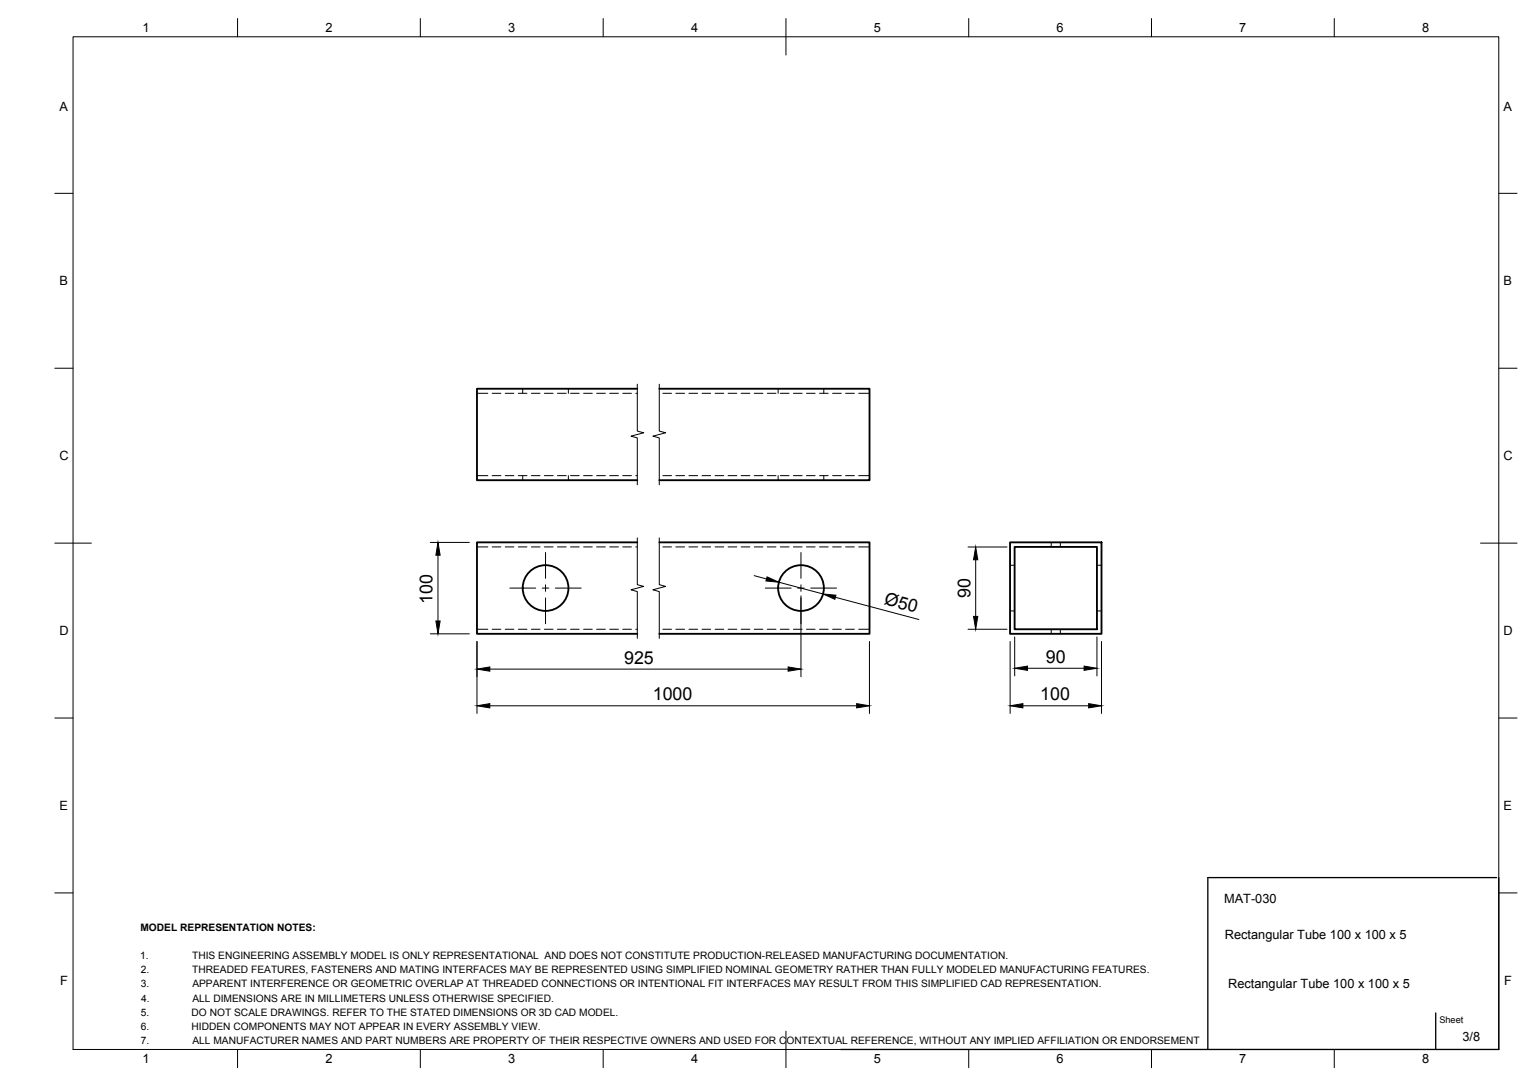
ISO-10303-21;
HEADER;
/* Generated by software containing ST-Developer
 * from STEP Tools, Inc. (www.steptools.com) 
 */

FILE_DESCRIPTION(
/* description */ ('STEP AP214'),
/* implementation_level */ '2;1');

FILE_NAME(
/* name */ 'Rectangular Tube 100 x 100 x 5.step',
/* time_stamp */ '2026-11-14T06:43:04-08:00',
/* author */ (''),
/* organization */ (''),
/* preprocessor_version */ 'ST-DEVELOPER v20.2',
/* originating_system */ 'Autodesk Translation Framework v15.17.0.0',
/* authorisation */ '');

FILE_SCHEMA (('AUTOMOTIVE_DESIGN { 1 0 10303 214 3 1 1 }'));
ENDSEC;

DATA;
#10=MECHANICAL_DESIGN_GEOMETRIC_PRESENTATION_REPRESENTATION('',(#204),#5658);
#182=SHAPE_REPRESENTATION_RELATIONSHIP('SRR','None',#5712,#193);
#193=ADVANCED_BREP_SHAPE_REPRESENTATION('',(#215),#5653);
#204=STYLED_ITEM('',(#5772),#215);
#215=MANIFOLD_SOLID_BREP('Body1',#3066);
#254=CYLINDRICAL_SURFACE('',#3398,5.);
#255=CYLINDRICAL_SURFACE('',#3401,5.);
#256=CYLINDRICAL_SURFACE('',#3404,5.);
#257=CYLINDRICAL_SURFACE('',#3407,5.);
#258=CYLINDRICAL_SURFACE('',#3410,25.);
#259=CYLINDRICAL_SURFACE('',#3413,25.);
#260=CYLINDRICAL_SURFACE('',#3416,25.);
#261=CYLINDRICAL_SURFACE('',#3419,25.);
#311=FACE_BOUND('',#675,.T.);
#312=FACE_BOUND('',#677,.T.);
#313=FACE_BOUND('',#679,.T.);
#314=FACE_BOUND('',#680,.T.);
#315=FACE_BOUND('',#682,.T.);
#316=FACE_BOUND('',#683,.T.);
#317=FACE_BOUND('',#685,.T.);
#318=FACE_BOUND('',#686,.T.);
#319=FACE_BOUND('',#688,.T.);
#320=FACE_BOUND('',#689,.T.);
#321=FACE_BOUND('',#691,.T.);
#322=FACE_BOUND('',#692,.T.);
#323=FACE_BOUND('',#694,.T.);
#324=FACE_BOUND('',#695,.T.);
#325=FACE_BOUND('',#697,.T.);
#326=FACE_BOUND('',#698,.T.);
#327=FACE_BOUND('',#700,.T.);
#328=FACE_BOUND('',#701,.T.);
#444=FACE_OUTER_BOUND('',#666,.T.);
#445=FACE_OUTER_BOUND('',#667,.T.);
#446=FACE_OUTER_BOUND('',#668,.T.);
#447=FACE_OUTER_BOUND('',#669,.T.);
#448=FACE_OUTER_BOUND('',#670,.T.);
#449=FACE_OUTER_BOUND('',#671,.T.);
#450=FACE_OUTER_BOUND('',#672,.T.);
#451=FACE_OUTER_BOUND('',#673,.T.);
#452=FACE_OUTER_BOUND('',#674,.T.);
#453=FACE_OUTER_BOUND('',#676,.T.);
#454=FACE_OUTER_BOUND('',#678,.T.);
#455=FACE_OUTER_BOUND('',#681,.T.);
#456=FACE_OUTER_BOUND('',#684,.T.);
#457=FACE_OUTER_BOUND('',#687,.T.);
#458=FACE_OUTER_BOUND('',#690,.T.);
#459=FACE_OUTER_BOUND('',#693,.T.);
#460=FACE_OUTER_BOUND('',#696,.T.);
#461=FACE_OUTER_BOUND('',#699,.T.);
#666=EDGE_LOOP('',(#2460,#2461,#2462,#2463));
#667=EDGE_LOOP('',(#2464,#2465,#2466,#2467));
#668=EDGE_LOOP('',(#2468,#2469,#2470,#2471));
#669=EDGE_LOOP('',(#2472,#2473,#2474,#2475));
#670=EDGE_LOOP('',(#2476,#2477,#2478,#2479));
#671=EDGE_LOOP('',(#2480,#2481,#2482,#2483));
#672=EDGE_LOOP('',(#2484,#2485,#2486,#2487));
#673=EDGE_LOOP('',(#2488,#2489,#2490,#2491));
#674=EDGE_LOOP('',(#2492,#2493,#2494,#2495));
#675=EDGE_LOOP('',(#2496,#2497,#2498,#2499));
#676=EDGE_LOOP('',(#2500,#2501,#2502,#2503));
#677=EDGE_LOOP('',(#2504,#2505,#2506,#2507));
#678=EDGE_LOOP('',(#2508,#2509,#2510,#2511));
#679=EDGE_LOOP('',(#2512));
#680=EDGE_LOOP('',(#2513));
#681=EDGE_LOOP('',(#2514,#2515,#2516,#2517));
#682=EDGE_LOOP('',(#2518));
#683=EDGE_LOOP('',(#2519));
#684=EDGE_LOOP('',(#2520,#2521,#2522,#2523));
#685=EDGE_LOOP('',(#2524));
#686=EDGE_LOOP('',(#2525));
#687=EDGE_LOOP('',(#2526,#2527,#2528,#2529));
#688=EDGE_LOOP('',(#2530));
#689=EDGE_LOOP('',(#2531));
#690=EDGE_LOOP('',(#2532,#2533,#2534,#2535));
#691=EDGE_LOOP('',(#2536));
#692=EDGE_LOOP('',(#2537));
#693=EDGE_LOOP('',(#2538,#2539,#2540,#2541));
#694=EDGE_LOOP('',(#2542));
#695=EDGE_LOOP('',(#2543));
#696=EDGE_LOOP('',(#2544,#2545,#2546,#2547));
#697=EDGE_LOOP('',(#2548));
#698=EDGE_LOOP('',(#2549));
#699=EDGE_LOOP('',(#2550,#2551,#2552,#2553));
#700=EDGE_LOOP('',(#2554));
#701=EDGE_LOOP('',(#2555));
#864=LINE('',#5273,#1060);
#865=LINE('',#5279,#1061);
#866=LINE('',#5285,#1062);
#867=LINE('',#5291,#1063);
#868=LINE('',#5297,#1064);
#869=LINE('',#5303,#1065);
#870=LINE('',#5309,#1066);
#871=LINE('',#5315,#1067);
#872=LINE('',#5320,#1068);
#873=LINE('',#5322,#1069);
#874=LINE('',#5324,#1070);
#875=LINE('',#5325,#1071);
#876=LINE('',#5328,#1072);
#877=LINE('',#5330,#1073);
#878=LINE('',#5332,#1074);
#879=LINE('',#5333,#1075);
#880=LINE('',#5337,#1076);
#881=LINE('',#5339,#1077);
#882=LINE('',#5341,#1078);
#883=LINE('',#5342,#1079);
#884=LINE('',#5345,#1080);
#885=LINE('',#5347,#1081);
#886=LINE('',#5349,#1082);
#887=LINE('',#5350,#1083);
#888=LINE('',#5352,#1084);
#889=LINE('',#5353,#1085);
#890=LINE('',#5355,#1086);
#891=LINE('',#5357,#1087);
#892=LINE('',#5360,#1088);
#893=LINE('',#5361,#1089);
#894=LINE('',#5363,#1090);
#895=LINE('',#5365,#1091);
#1060=VECTOR('',#4070,5.);
#1061=VECTOR('',#4077,5.);
#1062=VECTOR('',#4084,5.);
#1063=VECTOR('',#4091,5.);
#1064=VECTOR('',#4098,25.);
#1065=VECTOR('',#4105,25.);
#1066=VECTOR('',#4112,25.);
#1067=VECTOR('',#4119,25.);
#1068=VECTOR('',#4124,1000.);
#1069=VECTOR('',#4125,1000.);
#1070=VECTOR('',#4126,1000.);
#1071=VECTOR('',#4127,1000.);
#1072=VECTOR('',#4128,1000.);
#1073=VECTOR('',#4129,1000.);
#1074=VECTOR('',#4130,1000.);
#1075=VECTOR('',#4131,1000.);
#1076=VECTOR('',#4134,1000.);
#1077=VECTOR('',#4135,1000.);
#1078=VECTOR('',#4136,1000.);
#1079=VECTOR('',#4137,1000.);
#1080=VECTOR('',#4138,1000.);
#1081=VECTOR('',#4139,1000.);
#1082=VECTOR('',#4140,1000.);
#1083=VECTOR('',#4141,1000.);
#1084=VECTOR('',#4144,1000.);
#1085=VECTOR('',#4145,1000.);
#1086=VECTOR('',#4148,1000.);
#1087=VECTOR('',#4151,1000.);
#1088=VECTOR('',#4156,1000.);
#1089=VECTOR('',#4157,1000.);
#1090=VECTOR('',#4160,1000.);
#1091=VECTOR('',#4163,1000.);
#1250=CIRCLE('',#3399,5.);
#1251=CIRCLE('',#3400,5.);
#1252=CIRCLE('',#3402,5.);
#1253=CIRCLE('',#3403,5.);
#1254=CIRCLE('',#3405,5.);
#1255=CIRCLE('',#3406,5.);
#1256=CIRCLE('',#3408,5.);
#1257=CIRCLE('',#3409,5.);
#1258=CIRCLE('',#3411,25.);
#1259=CIRCLE('',#3412,25.);
#1260=CIRCLE('',#3414,25.);
#1261=CIRCLE('',#3415,25.);
#1262=CIRCLE('',#3417,25.);
#1263=CIRCLE('',#3418,25.);
#1264=CIRCLE('',#3420,25.);
#1265=CIRCLE('',#3421,25.);
#1467=VERTEX_POINT('',#5270);
#1468=VERTEX_POINT('',#5272);
#1469=VERTEX_POINT('',#5276);
#1470=VERTEX_POINT('',#5278);
#1471=VERTEX_POINT('',#5282);
#1472=VERTEX_POINT('',#5284);
#1473=VERTEX_POINT('',#5288);
#1474=VERTEX_POINT('',#5290);
#1475=VERTEX_POINT('',#5294);
#1476=VERTEX_POINT('',#5296);
#1477=VERTEX_POINT('',#5300);
#1478=VERTEX_POINT('',#5302);
#1479=VERTEX_POINT('',#5306);
#1480=VERTEX_POINT('',#5308);
#1481=VERTEX_POINT('',#5312);
#1482=VERTEX_POINT('',#5314);
#1483=VERTEX_POINT('',#5318);
#1484=VERTEX_POINT('',#5319);
#1485=VERTEX_POINT('',#5321);
#1486=VERTEX_POINT('',#5323);
#1487=VERTEX_POINT('',#5326);
#1488=VERTEX_POINT('',#5327);
#1489=VERTEX_POINT('',#5329);
#1490=VERTEX_POINT('',#5331);
#1491=VERTEX_POINT('',#5335);
#1492=VERTEX_POINT('',#5336);
#1493=VERTEX_POINT('',#5338);
#1494=VERTEX_POINT('',#5340);
#1495=VERTEX_POINT('',#5343);
#1496=VERTEX_POINT('',#5344);
#1497=VERTEX_POINT('',#5346);
#1498=VERTEX_POINT('',#5348);
#1813=EDGE_CURVE('',#1467,#1467,#1250,.T.);
#1814=EDGE_CURVE('',#1467,#1468,#864,.T.);
#1815=EDGE_CURVE('',#1468,#1468,#1251,.T.);
#1816=EDGE_CURVE('',#1469,#1469,#1252,.T.);
#1817=EDGE_CURVE('',#1469,#1470,#865,.T.);
#1818=EDGE_CURVE('',#1470,#1470,#1253,.T.);
#1819=EDGE_CURVE('',#1471,#1471,#1254,.T.);
#1820=EDGE_CURVE('',#1471,#1472,#866,.T.);
#1821=EDGE_CURVE('',#1472,#1472,#1255,.T.);
#1822=EDGE_CURVE('',#1473,#1473,#1256,.T.);
#1823=EDGE_CURVE('',#1473,#1474,#867,.T.);
#1824=EDGE_CURVE('',#1474,#1474,#1257,.T.);
#1825=EDGE_CURVE('',#1475,#1475,#1258,.T.);
#1826=EDGE_CURVE('',#1475,#1476,#868,.T.);
#1827=EDGE_CURVE('',#1476,#1476,#1259,.T.);
#1828=EDGE_CURVE('',#1477,#1477,#1260,.T.);
#1829=EDGE_CURVE('',#1477,#1478,#869,.T.);
#1830=EDGE_CURVE('',#1478,#1478,#1261,.T.);
#1831=EDGE_CURVE('',#1479,#1479,#1262,.T.);
#1832=EDGE_CURVE('',#1479,#1480,#870,.T.);
#1833=EDGE_CURVE('',#1480,#1480,#1263,.T.);
#1834=EDGE_CURVE('',#1481,#1481,#1264,.T.);
#1835=EDGE_CURVE('',#1481,#1482,#871,.T.);
#1836=EDGE_CURVE('',#1482,#1482,#1265,.T.);
#1837=EDGE_CURVE('',#1483,#1484,#872,.T.);
#1838=EDGE_CURVE('',#1484,#1485,#873,.T.);
#1839=EDGE_CURVE('',#1486,#1485,#874,.T.);
#1840=EDGE_CURVE('',#1483,#1486,#875,.T.);
#1841=EDGE_CURVE('',#1487,#1488,#876,.T.);
#1842=EDGE_CURVE('',#1489,#1487,#877,.T.);
#1843=EDGE_CURVE('',#1489,#1490,#878,.T.);
#1844=EDGE_CURVE('',#1490,#1488,#879,.T.);
#1845=EDGE_CURVE('',#1491,#1492,#880,.T.);
#1846=EDGE_CURVE('',#1491,#1493,#881,.T.);
#1847=EDGE_CURVE('',#1493,#1494,#882,.T.);
#1848=EDGE_CURVE('',#1492,#1494,#883,.T.);
#1849=EDGE_CURVE('',#1495,#1496,#884,.T.);
#1850=EDGE_CURVE('',#1496,#1497,#885,.T.);
#1851=EDGE_CURVE('',#1498,#1497,#886,.T.);
#1852=EDGE_CURVE('',#1495,#1498,#887,.T.);
#1853=EDGE_CURVE('',#1484,#1492,#888,.T.);
#1854=EDGE_CURVE('',#1483,#1491,#889,.T.);
#1855=EDGE_CURVE('',#1485,#1494,#890,.T.);
#1856=EDGE_CURVE('',#1486,#1493,#891,.T.);
#1857=EDGE_CURVE('',#1489,#1495,#892,.T.);
#1858=EDGE_CURVE('',#1487,#1496,#893,.T.);
#1859=EDGE_CURVE('',#1488,#1497,#894,.T.);
#1860=EDGE_CURVE('',#1490,#1498,#895,.T.);
#2460=ORIENTED_EDGE('',*,*,#1813,.F.);
#2461=ORIENTED_EDGE('',*,*,#1814,.T.);
#2462=ORIENTED_EDGE('',*,*,#1815,.T.);
#2463=ORIENTED_EDGE('',*,*,#1814,.F.);
#2464=ORIENTED_EDGE('',*,*,#1816,.F.);
#2465=ORIENTED_EDGE('',*,*,#1817,.T.);
#2466=ORIENTED_EDGE('',*,*,#1818,.T.);
#2467=ORIENTED_EDGE('',*,*,#1817,.F.);
#2468=ORIENTED_EDGE('',*,*,#1819,.F.);
#2469=ORIENTED_EDGE('',*,*,#1820,.T.);
#2470=ORIENTED_EDGE('',*,*,#1821,.T.);
#2471=ORIENTED_EDGE('',*,*,#1820,.F.);
#2472=ORIENTED_EDGE('',*,*,#1822,.F.);
#2473=ORIENTED_EDGE('',*,*,#1823,.T.);
#2474=ORIENTED_EDGE('',*,*,#1824,.T.);
#2475=ORIENTED_EDGE('',*,*,#1823,.F.);
#2476=ORIENTED_EDGE('',*,*,#1825,.T.);
#2477=ORIENTED_EDGE('',*,*,#1826,.T.);
#2478=ORIENTED_EDGE('',*,*,#1827,.T.);
#2479=ORIENTED_EDGE('',*,*,#1826,.F.);
#2480=ORIENTED_EDGE('',*,*,#1828,.T.);
#2481=ORIENTED_EDGE('',*,*,#1829,.T.);
#2482=ORIENTED_EDGE('',*,*,#1830,.T.);
#2483=ORIENTED_EDGE('',*,*,#1829,.F.);
#2484=ORIENTED_EDGE('',*,*,#1831,.F.);
#2485=ORIENTED_EDGE('',*,*,#1832,.T.);
#2486=ORIENTED_EDGE('',*,*,#1833,.F.);
#2487=ORIENTED_EDGE('',*,*,#1832,.F.);
#2488=ORIENTED_EDGE('',*,*,#1834,.F.);
#2489=ORIENTED_EDGE('',*,*,#1835,.T.);
#2490=ORIENTED_EDGE('',*,*,#1836,.F.);
#2491=ORIENTED_EDGE('',*,*,#1835,.F.);
#2492=ORIENTED_EDGE('',*,*,#1837,.T.);
#2493=ORIENTED_EDGE('',*,*,#1838,.T.);
#2494=ORIENTED_EDGE('',*,*,#1839,.F.);
#2495=ORIENTED_EDGE('',*,*,#1840,.F.);
#2496=ORIENTED_EDGE('',*,*,#1841,.F.);
#2497=ORIENTED_EDGE('',*,*,#1842,.F.);
#2498=ORIENTED_EDGE('',*,*,#1843,.T.);
#2499=ORIENTED_EDGE('',*,*,#1844,.T.);
#2500=ORIENTED_EDGE('',*,*,#1845,.F.);
#2501=ORIENTED_EDGE('',*,*,#1846,.T.);
#2502=ORIENTED_EDGE('',*,*,#1847,.T.);
#2503=ORIENTED_EDGE('',*,*,#1848,.F.);
#2504=ORIENTED_EDGE('',*,*,#1849,.T.);
#2505=ORIENTED_EDGE('',*,*,#1850,.T.);
#2506=ORIENTED_EDGE('',*,*,#1851,.F.);
#2507=ORIENTED_EDGE('',*,*,#1852,.F.);
#2508=ORIENTED_EDGE('',*,*,#1845,.T.);
#2509=ORIENTED_EDGE('',*,*,#1853,.F.);
#2510=ORIENTED_EDGE('',*,*,#1837,.F.);
#2511=ORIENTED_EDGE('',*,*,#1854,.T.);
#2512=ORIENTED_EDGE('',*,*,#1827,.F.);
#2513=ORIENTED_EDGE('',*,*,#1830,.F.);
#2514=ORIENTED_EDGE('',*,*,#1848,.T.);
#2515=ORIENTED_EDGE('',*,*,#1855,.F.);
#2516=ORIENTED_EDGE('',*,*,#1838,.F.);
#2517=ORIENTED_EDGE('',*,*,#1853,.T.);
#2518=ORIENTED_EDGE('',*,*,#1813,.T.);
#2519=ORIENTED_EDGE('',*,*,#1816,.T.);
#2520=ORIENTED_EDGE('',*,*,#1847,.F.);
#2521=ORIENTED_EDGE('',*,*,#1856,.F.);
#2522=ORIENTED_EDGE('',*,*,#1839,.T.);
#2523=ORIENTED_EDGE('',*,*,#1855,.T.);
#2524=ORIENTED_EDGE('',*,*,#1831,.T.);
#2525=ORIENTED_EDGE('',*,*,#1834,.T.);
#2526=ORIENTED_EDGE('',*,*,#1846,.F.);
#2527=ORIENTED_EDGE('',*,*,#1854,.F.);
#2528=ORIENTED_EDGE('',*,*,#1840,.T.);
#2529=ORIENTED_EDGE('',*,*,#1856,.T.);
#2530=ORIENTED_EDGE('',*,*,#1821,.F.);
#2531=ORIENTED_EDGE('',*,*,#1824,.F.);
#2532=ORIENTED_EDGE('',*,*,#1849,.F.);
#2533=ORIENTED_EDGE('',*,*,#1857,.F.);
#2534=ORIENTED_EDGE('',*,*,#1842,.T.);
#2535=ORIENTED_EDGE('',*,*,#1858,.T.);
#2536=ORIENTED_EDGE('',*,*,#1825,.F.);
#2537=ORIENTED_EDGE('',*,*,#1828,.F.);
#2538=ORIENTED_EDGE('',*,*,#1850,.F.);
#2539=ORIENTED_EDGE('',*,*,#1858,.F.);
#2540=ORIENTED_EDGE('',*,*,#1841,.T.);
#2541=ORIENTED_EDGE('',*,*,#1859,.T.);
#2542=ORIENTED_EDGE('',*,*,#1815,.F.);
#2543=ORIENTED_EDGE('',*,*,#1818,.F.);
#2544=ORIENTED_EDGE('',*,*,#1851,.T.);
#2545=ORIENTED_EDGE('',*,*,#1859,.F.);
#2546=ORIENTED_EDGE('',*,*,#1844,.F.);
#2547=ORIENTED_EDGE('',*,*,#1860,.T.);
#2548=ORIENTED_EDGE('',*,*,#1833,.T.);
#2549=ORIENTED_EDGE('',*,*,#1836,.T.);
#2550=ORIENTED_EDGE('',*,*,#1852,.T.);
#2551=ORIENTED_EDGE('',*,*,#1860,.F.);
#2552=ORIENTED_EDGE('',*,*,#1843,.F.);
#2553=ORIENTED_EDGE('',*,*,#1857,.T.);
#2554=ORIENTED_EDGE('',*,*,#1819,.T.);
#2555=ORIENTED_EDGE('',*,*,#1822,.T.);
#2832=PLANE('',#3422);
#2833=PLANE('',#3423);
#2834=PLANE('',#3424);
#2835=PLANE('',#3425);
#2836=PLANE('',#3426);
#2837=PLANE('',#3427);
#2838=PLANE('',#3428);
#2839=PLANE('',#3429);
#2840=PLANE('',#3430);
#2841=PLANE('',#3431);
#2985=ADVANCED_FACE('',(#444),#254,.F.);
#2986=ADVANCED_FACE('',(#445),#255,.F.);
#2987=ADVANCED_FACE('',(#446),#256,.F.);
#2988=ADVANCED_FACE('',(#447),#257,.F.);
#2989=ADVANCED_FACE('',(#448),#258,.F.);
#2990=ADVANCED_FACE('',(#449),#259,.F.);
#2991=ADVANCED_FACE('',(#450),#260,.F.);
#2992=ADVANCED_FACE('',(#451),#261,.F.);
#2993=ADVANCED_FACE('',(#452,#311),#2832,.T.);
#2994=ADVANCED_FACE('',(#453,#312),#2833,.F.);
#2995=ADVANCED_FACE('',(#454,#313,#314),#2834,.F.);
#2996=ADVANCED_FACE('',(#455,#315,#316),#2835,.F.);
#2997=ADVANCED_FACE('',(#456,#317,#318),#2836,.T.);
#2998=ADVANCED_FACE('',(#457,#319,#320),#2837,.T.);
#2999=ADVANCED_FACE('',(#458,#321,#322),#2838,.T.);
#3000=ADVANCED_FACE('',(#459,#323,#324),#2839,.T.);
#3001=ADVANCED_FACE('',(#460,#325,#326),#2840,.F.);
#3002=ADVANCED_FACE('',(#461,#327,#328),#2841,.F.);
#3066=CLOSED_SHELL('',(#2985,#2986,#2987,#2988,#2989,#2990,#2991,#2992,
#2993,#2994,#2995,#2996,#2997,#2998,#2999,#3000,#3001,#3002));
#3397=AXIS2_PLACEMENT_3D('',#5268,#4064,#4065);
#3398=AXIS2_PLACEMENT_3D('',#5269,#4066,#4067);
#3399=AXIS2_PLACEMENT_3D('',#5271,#4068,#4069);
#3400=AXIS2_PLACEMENT_3D('',#5274,#4071,#4072);
#3401=AXIS2_PLACEMENT_3D('',#5275,#4073,#4074);
#3402=AXIS2_PLACEMENT_3D('',#5277,#4075,#4076);
#3403=AXIS2_PLACEMENT_3D('',#5280,#4078,#4079);
#3404=AXIS2_PLACEMENT_3D('',#5281,#4080,#4081);
#3405=AXIS2_PLACEMENT_3D('',#5283,#4082,#4083);
#3406=AXIS2_PLACEMENT_3D('',#5286,#4085,#4086);
#3407=AXIS2_PLACEMENT_3D('',#5287,#4087,#4088);
#3408=AXIS2_PLACEMENT_3D('',#5289,#4089,#4090);
#3409=AXIS2_PLACEMENT_3D('',#5292,#4092,#4093);
#3410=AXIS2_PLACEMENT_3D('',#5293,#4094,#4095);
#3411=AXIS2_PLACEMENT_3D('',#5295,#4096,#4097);
#3412=AXIS2_PLACEMENT_3D('',#5298,#4099,#4100);
#3413=AXIS2_PLACEMENT_3D('',#5299,#4101,#4102);
#3414=AXIS2_PLACEMENT_3D('',#5301,#4103,#4104);
#3415=AXIS2_PLACEMENT_3D('',#5304,#4106,#4107);
#3416=AXIS2_PLACEMENT_3D('',#5305,#4108,#4109);
#3417=AXIS2_PLACEMENT_3D('',#5307,#4110,#4111);
#3418=AXIS2_PLACEMENT_3D('',#5310,#4113,#4114);
#3419=AXIS2_PLACEMENT_3D('',#5311,#4115,#4116);
#3420=AXIS2_PLACEMENT_3D('',#5313,#4117,#4118);
#3421=AXIS2_PLACEMENT_3D('',#5316,#4120,#4121);
#3422=AXIS2_PLACEMENT_3D('',#5317,#4122,#4123);
#3423=AXIS2_PLACEMENT_3D('',#5334,#4132,#4133);
#3424=AXIS2_PLACEMENT_3D('',#5351,#4142,#4143);
#3425=AXIS2_PLACEMENT_3D('',#5354,#4146,#4147);
#3426=AXIS2_PLACEMENT_3D('',#5356,#4149,#4150);
#3427=AXIS2_PLACEMENT_3D('',#5358,#4152,#4153);
#3428=AXIS2_PLACEMENT_3D('',#5359,#4154,#4155);
#3429=AXIS2_PLACEMENT_3D('',#5362,#4158,#4159);
#3430=AXIS2_PLACEMENT_3D('',#5364,#4161,#4162);
#3431=AXIS2_PLACEMENT_3D('',#5366,#4164,#4165);
#4064=DIRECTION('axis',(0.,0.,1.));
#4065=DIRECTION('refdir',(1.,0.,0.));
#4066=DIRECTION('center_axis',(0.,0.,1.));
#4067=DIRECTION('ref_axis',(1.,0.,0.));
#4068=DIRECTION('center_axis',(0.,0.,1.));
#4069=DIRECTION('ref_axis',(1.,0.,0.));
#4070=DIRECTION('',(0.,0.,1.));
#4071=DIRECTION('center_axis',(0.,0.,1.));
#4072=DIRECTION('ref_axis',(1.,0.,0.));
#4073=DIRECTION('center_axis',(0.,0.,1.));
#4074=DIRECTION('ref_axis',(1.,0.,0.));
#4075=DIRECTION('center_axis',(0.,0.,1.));
#4076=DIRECTION('ref_axis',(1.,0.,0.));
#4077=DIRECTION('',(0.,0.,1.));
#4078=DIRECTION('center_axis',(0.,0.,1.));
#4079=DIRECTION('ref_axis',(1.,0.,0.));
#4080=DIRECTION('center_axis',(0.,0.,1.));
#4081=DIRECTION('ref_axis',(1.,0.,0.));
#4082=DIRECTION('center_axis',(0.,0.,1.));
#4083=DIRECTION('ref_axis',(1.,0.,0.));
#4084=DIRECTION('',(0.,0.,1.));
#4085=DIRECTION('center_axis',(0.,0.,1.));
#4086=DIRECTION('ref_axis',(1.,0.,0.));
#4087=DIRECTION('center_axis',(0.,0.,1.));
#4088=DIRECTION('ref_axis',(1.,0.,0.));
#4089=DIRECTION('center_axis',(0.,0.,1.));
#4090=DIRECTION('ref_axis',(1.,0.,0.));
#4091=DIRECTION('',(0.,0.,1.));
#4092=DIRECTION('center_axis',(0.,0.,1.));
#4093=DIRECTION('ref_axis',(1.,0.,0.));
#4094=DIRECTION('center_axis',(1.,0.,-6.93889390390723E-17));
#4095=DIRECTION('ref_axis',(-6.93889390390723E-17,0.,-1.));
#4096=DIRECTION('center_axis',(-1.,0.,6.93889390390723E-17));
#4097=DIRECTION('ref_axis',(6.93889390390723E-17,0.,1.));
#4098=DIRECTION('',(1.,0.,-6.93889390390723E-17));
#4099=DIRECTION('center_axis',(1.,0.,-6.93889390390723E-17));
#4100=DIRECTION('ref_axis',(-6.93889390390723E-17,0.,-1.));
#4101=DIRECTION('center_axis',(1.,0.,-6.93889390390723E-17));
#4102=DIRECTION('ref_axis',(-6.93889390390723E-17,0.,-1.));
#4103=DIRECTION('center_axis',(-1.,0.,6.93889390390723E-17));
#4104=DIRECTION('ref_axis',(6.93889390390723E-17,0.,1.));
#4105=DIRECTION('',(1.,0.,-6.93889390390723E-17));
#4106=DIRECTION('center_axis',(1.,0.,-6.93889390390723E-17));
#4107=DIRECTION('ref_axis',(6.93889390390723E-17,0.,1.));
#4108=DIRECTION('center_axis',(1.,0.,-6.93889390390723E-17));
#4109=DIRECTION('ref_axis',(-6.93889390390723E-17,0.,-1.));
#4110=DIRECTION('center_axis',(1.,0.,-6.93889390390723E-17));
#4111=DIRECTION('ref_axis',(-6.93889390390723E-17,0.,-1.));
#4112=DIRECTION('',(1.,0.,-6.93889390390723E-17));
#4113=DIRECTION('center_axis',(-1.,0.,-6.93889390390723E-17));
#4114=DIRECTION('ref_axis',(-6.93889390390723E-17,0.,1.));
#4115=DIRECTION('center_axis',(1.,0.,-6.93889390390723E-17));
#4116=DIRECTION('ref_axis',(-6.93889390390723E-17,0.,-1.));
#4117=DIRECTION('center_axis',(1.,0.,-6.93889390390723E-17));
#4118=DIRECTION('ref_axis',(6.93889390390723E-17,0.,1.));
#4119=DIRECTION('',(1.,0.,-6.93889390390723E-17));
#4120=DIRECTION('center_axis',(-1.,0.,-6.93889390390723E-17));
#4121=DIRECTION('ref_axis',(-6.93889390390723E-17,0.,1.));
#4122=DIRECTION('center_axis',(0.,1.,0.));
#4123=DIRECTION('ref_axis',(0.,0.,1.));
#4124=DIRECTION('',(-6.93889390390723E-17,0.,-1.));
#4125=DIRECTION('',(-1.,0.,0.));
#4126=DIRECTION('',(6.93889390390723E-17,0.,-1.));
#4127=DIRECTION('',(-1.,0.,0.));
#4128=DIRECTION('',(-1.,0.,0.));
#4129=DIRECTION('',(-6.93889390390723E-17,0.,-1.));
#4130=DIRECTION('',(-1.,0.,0.));
#4131=DIRECTION('',(6.93889390390723E-17,0.,-1.));
#4132=DIRECTION('center_axis',(0.,1.,0.));
#4133=DIRECTION('ref_axis',(0.,0.,1.));
#4134=DIRECTION('',(-6.93889390390723E-17,0.,-1.));
#4135=DIRECTION('',(-1.,0.,0.));
#4136=DIRECTION('',(6.93889390390723E-17,0.,-1.));
#4137=DIRECTION('',(-1.,0.,0.));
#4138=DIRECTION('',(-6.93889390390723E-17,0.,-1.));
#4139=DIRECTION('',(-1.,0.,0.));
#4140=DIRECTION('',(6.93889390390723E-17,0.,-1.));
#4141=DIRECTION('',(-1.,0.,0.));
#4142=DIRECTION('center_axis',(-1.,0.,6.93889390390723E-17));
#4143=DIRECTION('ref_axis',(6.93889390390723E-17,0.,1.));
#4144=DIRECTION('',(0.,-1.,0.));
#4145=DIRECTION('',(0.,-1.,0.));
#4146=DIRECTION('center_axis',(0.,0.,1.));
#4147=DIRECTION('ref_axis',(1.,0.,0.));
#4148=DIRECTION('',(0.,-1.,0.));
#4149=DIRECTION('center_axis',(-1.,0.,-6.93889390390723E-17));
#4150=DIRECTION('ref_axis',(-6.93889390390723E-17,0.,1.));
#4151=DIRECTION('',(0.,-1.,0.));
#4152=DIRECTION('center_axis',(0.,0.,1.));
#4153=DIRECTION('ref_axis',(1.,0.,0.));
#4154=DIRECTION('center_axis',(-1.,0.,6.93889390390723E-17));
#4155=DIRECTION('ref_axis',(6.93889390390723E-17,0.,1.));
#4156=DIRECTION('',(0.,-1.,0.));
#4157=DIRECTION('',(0.,-1.,0.));
#4158=DIRECTION('center_axis',(0.,0.,1.));
#4159=DIRECTION('ref_axis',(1.,0.,0.));
#4160=DIRECTION('',(0.,-1.,0.));
#4161=DIRECTION('center_axis',(-1.,0.,-6.93889390390723E-17));
#4162=DIRECTION('ref_axis',(-6.93889390390723E-17,0.,1.));
#4163=DIRECTION('',(0.,-1.,0.));
#4164=DIRECTION('center_axis',(0.,0.,1.));
#4165=DIRECTION('ref_axis',(1.,0.,0.));
#5268=CARTESIAN_POINT('',(0.,0.,0.));
#5269=CARTESIAN_POINT('Origin',(0.,30.,-50.));
#5270=CARTESIAN_POINT('',(-5.,30.,-50.));
#5271=CARTESIAN_POINT('Origin',(0.,30.,-50.));
#5272=CARTESIAN_POINT('',(-5.,30.,-45.));
#5273=CARTESIAN_POINT('',(-5.,30.,-50.));
#5274=CARTESIAN_POINT('Origin',(0.,30.,-45.));
#5275=CARTESIAN_POINT('Origin',(0.,-30.,-50.));
#5276=CARTESIAN_POINT('',(-5.,-30.,-50.));
#5277=CARTESIAN_POINT('Origin',(0.,-30.,-50.));
#5278=CARTESIAN_POINT('',(-5.,-30.,-45.));
#5279=CARTESIAN_POINT('',(-5.,-30.,-50.));
#5280=CARTESIAN_POINT('Origin',(0.,-30.,-45.));
#5281=CARTESIAN_POINT('Origin',(0.,30.,-50.));
#5282=CARTESIAN_POINT('',(-5.,30.,45.));
#5283=CARTESIAN_POINT('Origin',(0.,30.,45.));
#5284=CARTESIAN_POINT('',(-5.,30.,50.));
#5285=CARTESIAN_POINT('',(-5.,30.,-50.));
#5286=CARTESIAN_POINT('Origin',(0.,30.,50.));
#5287=CARTESIAN_POINT('Origin',(0.,-30.,-50.));
#5288=CARTESIAN_POINT('',(-5.,-30.,45.));
#5289=CARTESIAN_POINT('Origin',(0.,-30.,45.));
#5290=CARTESIAN_POINT('',(-5.,-30.,50.));
#5291=CARTESIAN_POINT('',(-5.,-30.,-50.));
#5292=CARTESIAN_POINT('Origin',(0.,-30.,50.));
#5293=CARTESIAN_POINT('Origin',(-50.,-425.,3.46944695195361E-15));
#5294=CARTESIAN_POINT('',(45.,-425.,25.));
#5295=CARTESIAN_POINT('Origin',(45.,-425.,-3.12250225675825E-15));
#5296=CARTESIAN_POINT('',(50.,-425.,25.));
#5297=CARTESIAN_POINT('',(-50.,-425.,25.));
#5298=CARTESIAN_POINT('Origin',(50.,-425.,-3.46944695195361E-15));
#5299=CARTESIAN_POINT('Origin',(-50.,425.,3.46944695195361E-15));
#5300=CARTESIAN_POINT('',(45.,425.,25.));
#5301=CARTESIAN_POINT('Origin',(45.,425.,-3.12250225675825E-15));
#5302=CARTESIAN_POINT('',(50.,425.,25.));
#5303=CARTESIAN_POINT('',(-50.,425.,25.));
#5304=CARTESIAN_POINT('Origin',(50.,425.,-3.46944695195361E-15));
#5305=CARTESIAN_POINT('Origin',(-50.,-425.,3.46944695195361E-15));
#5306=CARTESIAN_POINT('',(-50.,-425.,25.));
#5307=CARTESIAN_POINT('Origin',(-50.,-425.,3.46944695195361E-15));
#5308=CARTESIAN_POINT('',(-45.,-425.,25.));
#5309=CARTESIAN_POINT('',(-50.,-425.,25.));
#5310=CARTESIAN_POINT('Origin',(-45.,-425.,3.12250225675825E-15));
#5311=CARTESIAN_POINT('Origin',(-50.,425.,3.46944695195361E-15));
#5312=CARTESIAN_POINT('',(-50.,425.,25.));
#5313=CARTESIAN_POINT('Origin',(-50.,425.,3.46944695195361E-15));
#5314=CARTESIAN_POINT('',(-45.,425.,25.));
#5315=CARTESIAN_POINT('',(-50.,425.,25.));
#5316=CARTESIAN_POINT('Origin',(-45.,425.,3.12250225675825E-15));
#5317=CARTESIAN_POINT('Origin',(0.,500.,0.));
#5318=CARTESIAN_POINT('',(50.,500.,50.));
#5319=CARTESIAN_POINT('',(50.,500.,-50.));
#5320=CARTESIAN_POINT('',(50.,500.,50.));
#5321=CARTESIAN_POINT('',(-50.,500.,-50.));
#5322=CARTESIAN_POINT('',(50.,500.,-50.));
#5323=CARTESIAN_POINT('',(-50.,500.,50.));
#5324=CARTESIAN_POINT('',(-50.,500.,50.));
#5325=CARTESIAN_POINT('',(50.,500.,50.));
#5326=CARTESIAN_POINT('',(45.,500.,-45.));
#5327=CARTESIAN_POINT('',(-45.,500.,-45.));
#5328=CARTESIAN_POINT('',(50.,500.,-45.));
#5329=CARTESIAN_POINT('',(45.,500.,45.));
#5330=CARTESIAN_POINT('',(45.,500.,50.));
#5331=CARTESIAN_POINT('',(-45.,500.,45.));
#5332=CARTESIAN_POINT('',(50.,500.,45.));
#5333=CARTESIAN_POINT('',(-45.,500.,50.));
#5334=CARTESIAN_POINT('Origin',(0.,-500.,0.));
#5335=CARTESIAN_POINT('',(50.,-500.,50.));
#5336=CARTESIAN_POINT('',(50.,-500.,-50.));
#5337=CARTESIAN_POINT('',(50.,-500.,50.));
#5338=CARTESIAN_POINT('',(-50.,-500.,50.));
#5339=CARTESIAN_POINT('',(50.,-500.,50.));
#5340=CARTESIAN_POINT('',(-50.,-500.,-50.));
#5341=CARTESIAN_POINT('',(-50.,-500.,50.));
#5342=CARTESIAN_POINT('',(50.,-500.,-50.));
#5343=CARTESIAN_POINT('',(45.,-500.,45.));
#5344=CARTESIAN_POINT('',(45.,-500.,-45.));
#5345=CARTESIAN_POINT('',(45.,-500.,50.));
#5346=CARTESIAN_POINT('',(-45.,-500.,-45.));
#5347=CARTESIAN_POINT('',(50.,-500.,-45.));
#5348=CARTESIAN_POINT('',(-45.,-500.,45.));
#5349=CARTESIAN_POINT('',(-45.,-500.,50.));
#5350=CARTESIAN_POINT('',(50.,-500.,45.));
#5351=CARTESIAN_POINT('Origin',(50.,500.,50.));
#5352=CARTESIAN_POINT('',(50.,500.,-50.));
#5353=CARTESIAN_POINT('',(50.,500.,50.));
#5354=CARTESIAN_POINT('Origin',(50.,500.,-50.));
#5355=CARTESIAN_POINT('',(-50.,500.,-50.));
#5356=CARTESIAN_POINT('Origin',(-50.,500.,50.));
#5357=CARTESIAN_POINT('',(-50.,500.,50.));
#5358=CARTESIAN_POINT('Origin',(50.,500.,50.));
#5359=CARTESIAN_POINT('Origin',(45.,500.,50.));
#5360=CARTESIAN_POINT('',(45.,500.,45.));
#5361=CARTESIAN_POINT('',(45.,500.,-45.));
#5362=CARTESIAN_POINT('Origin',(50.,500.,-45.));
#5363=CARTESIAN_POINT('',(-45.,500.,-45.));
#5364=CARTESIAN_POINT('Origin',(-45.,500.,50.));
#5365=CARTESIAN_POINT('',(-45.,500.,45.));
#5366=CARTESIAN_POINT('Origin',(50.,500.,45.));
#5640=UNCERTAINTY_MEASURE_WITH_UNIT(LENGTH_MEASURE(0.01),#5659,
'DISTANCE_ACCURACY_VALUE',
'Maximum model space distance between geometric entities at asserted c
onnectivities');
#5645=UNCERTAINTY_MEASURE_WITH_UNIT(LENGTH_MEASURE(0.01),#5659,
'DISTANCE_ACCURACY_VALUE',
'Maximum model space distance between geometric entities at asserted c
onnectivities');
#5653=(
GEOMETRIC_REPRESENTATION_CONTEXT(3)
GLOBAL_UNCERTAINTY_ASSIGNED_CONTEXT((#5640))
GLOBAL_UNIT_ASSIGNED_CONTEXT((#5659,#5661,#5662))
REPRESENTATION_CONTEXT('','3D')
);
#5658=(
GEOMETRIC_REPRESENTATION_CONTEXT(3)
GLOBAL_UNCERTAINTY_ASSIGNED_CONTEXT((#5645))
GLOBAL_UNIT_ASSIGNED_CONTEXT((#5659,#5661,#5662))
REPRESENTATION_CONTEXT('','3D')
);
#5659=(
LENGTH_UNIT()
NAMED_UNIT(*)
SI_UNIT(.MILLI.,.METRE.)
);
#5661=(
NAMED_UNIT(*)
PLANE_ANGLE_UNIT()
SI_UNIT($,.RADIAN.)
);
#5662=(
NAMED_UNIT(*)
SI_UNIT($,.STERADIAN.)
SOLID_ANGLE_UNIT()
);
#5670=SHAPE_DEFINITION_REPRESENTATION(#5682,#5712);
#5682=PRODUCT_DEFINITION_SHAPE('',$,#5725);
#5712=SHAPE_REPRESENTATION('',(#3397),#5653);
#5717=PRODUCT_DEFINITION_CONTEXT('part definition',#5755,'design');
#5725=PRODUCT_DEFINITION('Rectangular Tube 100 x 100 x 5',
'Rectangular Tube 100 x 100 x 5',#5737,#5717);
#5737=PRODUCT_DEFINITION_FORMATION('',$,#5764);
#5755=APPLICATION_CONTEXT(
'Core Data for Automotive Mechanical Design Process');
#5756=PRODUCT_CONTEXT('part definition',#5755,'mechanical');
#5764=PRODUCT('Rectangular Tube 100 x 100 x 5',
'Rectangular Tube 100 x 100 x 5',$,(#5756));
#5772=PRESENTATION_STYLE_ASSIGNMENT((#5777));
#5777=SURFACE_STYLE_USAGE(.BOTH.,#5782);
#5782=SURFACE_SIDE_STYLE('',(#5787));
#5787=SURFACE_STYLE_FILL_AREA(#5792);
#5792=FILL_AREA_STYLE('Opaque(227,224,212)',(#5797));
#5797=FILL_AREA_STYLE_COLOUR('Opaque(227,224,212)',#5802);
#5802=COLOUR_RGB('Opaque(227,224,212)',0.890196078431372,0.87843137254902,
0.831372549019608);
ENDSEC;
END-ISO-10303-21;
